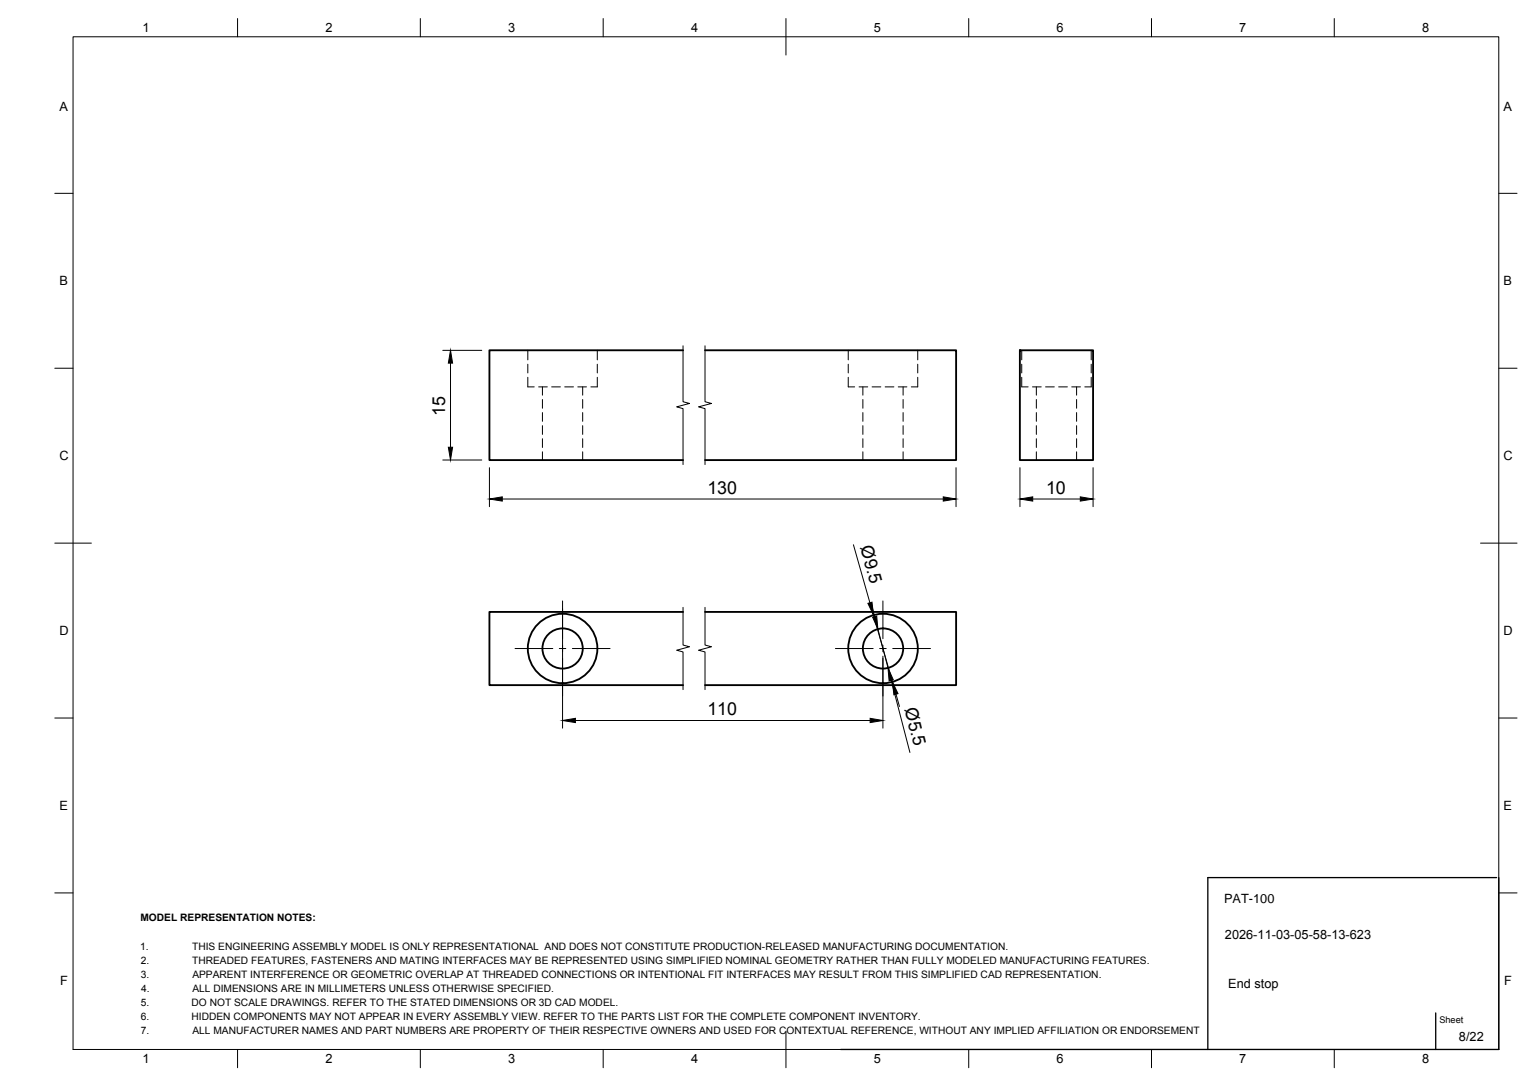
ISO-10303-21;
HEADER;
/* Generated by software containing ST-Developer
 * from STEP Tools, Inc. (www.steptools.com) 
 */

FILE_DESCRIPTION(
/* description */ (''),
/* implementation_level */ '2;1');

FILE_NAME(
/* name */ 'End stop.step',
/* time_stamp */ '2026-10-29T16:43:51-07:00',
/* author */ (''),
/* organization */ (''),
/* preprocessor_version */ 'ST-DEVELOPER v20.2',
/* originating_system */ 'Autodesk Translation Framework v15.17.0.0',
/* authorisation */ '');

FILE_SCHEMA (('AUTOMOTIVE_DESIGN { 1 0 10303 214 3 1 1 }'));
ENDSEC;

DATA;
#10=MECHANICAL_DESIGN_GEOMETRIC_PRESENTATION_REPRESENTATION('',(#369),#10292);
#323=SHAPE_REPRESENTATION_RELATIONSHIP('SRR','None',#10419,#346);
#346=ADVANCED_BREP_SHAPE_REPRESENTATION('',(#391),#10271);
#369=STYLED_ITEM('',(#10621),#391);
#391=MANIFOLD_SOLID_BREP('Body1',#5012);
#449=FACE_BOUND('',#1109,.T.);
#450=FACE_BOUND('',#1112,.T.);
#451=FACE_BOUND('',#1120,.T.);
#452=FACE_BOUND('',#1121,.T.);
#453=FACE_BOUND('',#1123,.T.);
#454=FACE_BOUND('',#1124,.T.);
#566=PLANE('',#5422);
#567=PLANE('',#5427);
#568=PLANE('',#5433);
#569=PLANE('',#5434);
#570=PLANE('',#5435);
#571=PLANE('',#5436);
#572=PLANE('',#5437);
#573=PLANE('',#5438);
#776=FACE_OUTER_BOUND('',#1107,.T.);
#777=FACE_OUTER_BOUND('',#1108,.T.);
#778=FACE_OUTER_BOUND('',#1110,.T.);
#779=FACE_OUTER_BOUND('',#1111,.T.);
#780=FACE_OUTER_BOUND('',#1113,.T.);
#781=FACE_OUTER_BOUND('',#1114,.T.);
#782=FACE_OUTER_BOUND('',#1115,.T.);
#783=FACE_OUTER_BOUND('',#1116,.T.);
#784=FACE_OUTER_BOUND('',#1117,.T.);
#785=FACE_OUTER_BOUND('',#1118,.T.);
#786=FACE_OUTER_BOUND('',#1119,.T.);
#787=FACE_OUTER_BOUND('',#1122,.T.);
#1107=EDGE_LOOP('',(#3729,#3730,#3731,#3732));
#1108=EDGE_LOOP('',(#3733));
#1109=EDGE_LOOP('',(#3734));
#1110=EDGE_LOOP('',(#3735,#3736,#3737,#3738));
#1111=EDGE_LOOP('',(#3739));
#1112=EDGE_LOOP('',(#3740));
#1113=EDGE_LOOP('',(#3741,#3742,#3743,#3744));
#1114=EDGE_LOOP('',(#3745,#3746,#3747,#3748));
#1115=EDGE_LOOP('',(#3749,#3750,#3751,#3752));
#1116=EDGE_LOOP('',(#3753,#3754,#3755,#3756));
#1117=EDGE_LOOP('',(#3757,#3758,#3759,#3760));
#1118=EDGE_LOOP('',(#3761,#3762,#3763,#3764));
#1119=EDGE_LOOP('',(#3765,#3766,#3767,#3768));
#1120=EDGE_LOOP('',(#3769));
#1121=EDGE_LOOP('',(#3770));
#1122=EDGE_LOOP('',(#3771,#3772,#3773,#3774));
#1123=EDGE_LOOP('',(#3775));
#1124=EDGE_LOOP('',(#3776));
#1514=LINE('',#7748,#1906);
#1515=LINE('',#7757,#1907);
#1516=LINE('',#7765,#1908);
#1517=LINE('',#7769,#1909);
#1518=LINE('',#7773,#1910);
#1519=LINE('',#7775,#1911);
#1520=LINE('',#7777,#1912);
#1521=LINE('',#7778,#1913);
#1522=LINE('',#7781,#1914);
#1523=LINE('',#7783,#1915);
#1524=LINE('',#7784,#1916);
#1525=LINE('',#7787,#1917);
#1526=LINE('',#7789,#1918);
#1527=LINE('',#7790,#1919);
#1528=LINE('',#7792,#1920);
#1529=LINE('',#7793,#1921);
#1906=VECTOR('',#6231,0.475);
#1907=VECTOR('',#6242,0.475);
#1908=VECTOR('',#6253,0.275);
#1909=VECTOR('',#6258,0.275);
#1910=VECTOR('',#6261,1.);
#1911=VECTOR('',#6262,1.);
#1912=VECTOR('',#6263,1.);
#1913=VECTOR('',#6264,1.);
#1914=VECTOR('',#6267,1.);
#1915=VECTOR('',#6268,1.);
#1916=VECTOR('',#6269,1.);
#1917=VECTOR('',#6272,1.);
#1918=VECTOR('',#6273,1.);
#1919=VECTOR('',#6274,1.);
#1920=VECTOR('',#6277,1.);
#1921=VECTOR('',#6278,1.);
#2252=CIRCLE('',#5420,0.475);
#2253=CIRCLE('',#5421,0.475);
#2254=CIRCLE('',#5423,0.275);
#2255=CIRCLE('',#5425,0.475);
#2256=CIRCLE('',#5426,0.475);
#2257=CIRCLE('',#5428,0.275);
#2258=CIRCLE('',#5430,0.275);
#2259=CIRCLE('',#5432,0.275);
#2499=VERTEX_POINT('',#7745);
#2500=VERTEX_POINT('',#7747);
#2501=VERTEX_POINT('',#7751);
#2502=VERTEX_POINT('',#7754);
#2503=VERTEX_POINT('',#7756);
#2504=VERTEX_POINT('',#7760);
#2505=VERTEX_POINT('',#7763);
#2506=VERTEX_POINT('',#7767);
#2507=VERTEX_POINT('',#7771);
#2508=VERTEX_POINT('',#7772);
#2509=VERTEX_POINT('',#7774);
#2510=VERTEX_POINT('',#7776);
#2511=VERTEX_POINT('',#7780);
#2512=VERTEX_POINT('',#7782);
#2513=VERTEX_POINT('',#7786);
#2514=VERTEX_POINT('',#7788);
#2955=EDGE_CURVE('',#2499,#2499,#2252,.T.);
#2956=EDGE_CURVE('',#2499,#2500,#1514,.T.);
#2957=EDGE_CURVE('',#2500,#2500,#2253,.T.);
#2958=EDGE_CURVE('',#2501,#2501,#2254,.T.);
#2959=EDGE_CURVE('',#2502,#2502,#2255,.T.);
#2960=EDGE_CURVE('',#2502,#2503,#1515,.T.);
#2961=EDGE_CURVE('',#2503,#2503,#2256,.T.);
#2962=EDGE_CURVE('',#2504,#2504,#2257,.T.);
#2963=EDGE_CURVE('',#2505,#2505,#2258,.T.);
#2964=EDGE_CURVE('',#2505,#2501,#1516,.T.);
#2965=EDGE_CURVE('',#2506,#2506,#2259,.T.);
#2966=EDGE_CURVE('',#2506,#2504,#1517,.T.);
#2967=EDGE_CURVE('',#2507,#2508,#1518,.T.);
#2968=EDGE_CURVE('',#2508,#2509,#1519,.T.);
#2969=EDGE_CURVE('',#2510,#2509,#1520,.T.);
#2970=EDGE_CURVE('',#2507,#2510,#1521,.T.);
#2971=EDGE_CURVE('',#2511,#2507,#1522,.T.);
#2972=EDGE_CURVE('',#2512,#2510,#1523,.T.);
#2973=EDGE_CURVE('',#2511,#2512,#1524,.T.);
#2974=EDGE_CURVE('',#2513,#2511,#1525,.T.);
#2975=EDGE_CURVE('',#2514,#2512,#1526,.T.);
#2976=EDGE_CURVE('',#2513,#2514,#1527,.T.);
#2977=EDGE_CURVE('',#2508,#2513,#1528,.T.);
#2978=EDGE_CURVE('',#2509,#2514,#1529,.T.);
#3729=ORIENTED_EDGE('',*,*,#2955,.F.);
#3730=ORIENTED_EDGE('',*,*,#2956,.T.);
#3731=ORIENTED_EDGE('',*,*,#2957,.F.);
#3732=ORIENTED_EDGE('',*,*,#2956,.F.);
#3733=ORIENTED_EDGE('',*,*,#2955,.T.);
#3734=ORIENTED_EDGE('',*,*,#2958,.F.);
#3735=ORIENTED_EDGE('',*,*,#2959,.F.);
#3736=ORIENTED_EDGE('',*,*,#2960,.T.);
#3737=ORIENTED_EDGE('',*,*,#2961,.F.);
#3738=ORIENTED_EDGE('',*,*,#2960,.F.);
#3739=ORIENTED_EDGE('',*,*,#2959,.T.);
#3740=ORIENTED_EDGE('',*,*,#2962,.F.);
#3741=ORIENTED_EDGE('',*,*,#2963,.F.);
#3742=ORIENTED_EDGE('',*,*,#2964,.T.);
#3743=ORIENTED_EDGE('',*,*,#2958,.T.);
#3744=ORIENTED_EDGE('',*,*,#2964,.F.);
#3745=ORIENTED_EDGE('',*,*,#2965,.F.);
#3746=ORIENTED_EDGE('',*,*,#2966,.T.);
#3747=ORIENTED_EDGE('',*,*,#2962,.T.);
#3748=ORIENTED_EDGE('',*,*,#2966,.F.);
#3749=ORIENTED_EDGE('',*,*,#2967,.T.);
#3750=ORIENTED_EDGE('',*,*,#2968,.T.);
#3751=ORIENTED_EDGE('',*,*,#2969,.F.);
#3752=ORIENTED_EDGE('',*,*,#2970,.F.);
#3753=ORIENTED_EDGE('',*,*,#2971,.T.);
#3754=ORIENTED_EDGE('',*,*,#2970,.T.);
#3755=ORIENTED_EDGE('',*,*,#2972,.F.);
#3756=ORIENTED_EDGE('',*,*,#2973,.F.);
#3757=ORIENTED_EDGE('',*,*,#2974,.T.);
#3758=ORIENTED_EDGE('',*,*,#2973,.T.);
#3759=ORIENTED_EDGE('',*,*,#2975,.F.);
#3760=ORIENTED_EDGE('',*,*,#2976,.F.);
#3761=ORIENTED_EDGE('',*,*,#2977,.T.);
#3762=ORIENTED_EDGE('',*,*,#2976,.T.);
#3763=ORIENTED_EDGE('',*,*,#2978,.F.);
#3764=ORIENTED_EDGE('',*,*,#2968,.F.);
#3765=ORIENTED_EDGE('',*,*,#2978,.T.);
#3766=ORIENTED_EDGE('',*,*,#2975,.T.);
#3767=ORIENTED_EDGE('',*,*,#2972,.T.);
#3768=ORIENTED_EDGE('',*,*,#2969,.T.);
#3769=ORIENTED_EDGE('',*,*,#2957,.T.);
#3770=ORIENTED_EDGE('',*,*,#2961,.T.);
#3771=ORIENTED_EDGE('',*,*,#2977,.F.);
#3772=ORIENTED_EDGE('',*,*,#2967,.F.);
#3773=ORIENTED_EDGE('',*,*,#2971,.F.);
#3774=ORIENTED_EDGE('',*,*,#2974,.F.);
#3775=ORIENTED_EDGE('',*,*,#2963,.T.);
#3776=ORIENTED_EDGE('',*,*,#2965,.T.);
#4663=CYLINDRICAL_SURFACE('',#5419,0.475);
#4664=CYLINDRICAL_SURFACE('',#5424,0.475);
#4665=CYLINDRICAL_SURFACE('',#5429,0.275);
#4666=CYLINDRICAL_SURFACE('',#5431,0.275);
#4785=ADVANCED_FACE('',(#776),#4663,.F.);
#4786=ADVANCED_FACE('',(#777,#449),#566,.T.);
#4787=ADVANCED_FACE('',(#778),#4664,.F.);
#4788=ADVANCED_FACE('',(#779,#450),#567,.T.);
#4789=ADVANCED_FACE('',(#780),#4665,.F.);
#4790=ADVANCED_FACE('',(#781),#4666,.F.);
#4791=ADVANCED_FACE('',(#782),#568,.T.);
#4792=ADVANCED_FACE('',(#783),#569,.T.);
#4793=ADVANCED_FACE('',(#784),#570,.T.);
#4794=ADVANCED_FACE('',(#785),#571,.T.);
#4795=ADVANCED_FACE('',(#786,#451,#452),#572,.T.);
#4796=ADVANCED_FACE('',(#787,#453,#454),#573,.F.);
#5012=CLOSED_SHELL('',(#4785,#4786,#4787,#4788,#4789,#4790,#4791,#4792,
#4793,#4794,#4795,#4796));
#5418=AXIS2_PLACEMENT_3D('',#7743,#6225,#6226);
#5419=AXIS2_PLACEMENT_3D('',#7744,#6227,#6228);
#5420=AXIS2_PLACEMENT_3D('',#7746,#6229,#6230);
#5421=AXIS2_PLACEMENT_3D('',#7749,#6232,#6233);
#5422=AXIS2_PLACEMENT_3D('',#7750,#6234,#6235);
#5423=AXIS2_PLACEMENT_3D('',#7752,#6236,#6237);
#5424=AXIS2_PLACEMENT_3D('',#7753,#6238,#6239);
#5425=AXIS2_PLACEMENT_3D('',#7755,#6240,#6241);
#5426=AXIS2_PLACEMENT_3D('',#7758,#6243,#6244);
#5427=AXIS2_PLACEMENT_3D('',#7759,#6245,#6246);
#5428=AXIS2_PLACEMENT_3D('',#7761,#6247,#6248);
#5429=AXIS2_PLACEMENT_3D('',#7762,#6249,#6250);
#5430=AXIS2_PLACEMENT_3D('',#7764,#6251,#6252);
#5431=AXIS2_PLACEMENT_3D('',#7766,#6254,#6255);
#5432=AXIS2_PLACEMENT_3D('',#7768,#6256,#6257);
#5433=AXIS2_PLACEMENT_3D('',#7770,#6259,#6260);
#5434=AXIS2_PLACEMENT_3D('',#7779,#6265,#6266);
#5435=AXIS2_PLACEMENT_3D('',#7785,#6270,#6271);
#5436=AXIS2_PLACEMENT_3D('',#7791,#6275,#6276);
#5437=AXIS2_PLACEMENT_3D('',#7794,#6279,#6280);
#5438=AXIS2_PLACEMENT_3D('',#7795,#6281,#6282);
#6225=DIRECTION('axis',(0.,0.,1.));
#6226=DIRECTION('refdir',(1.,0.,0.));
#6227=DIRECTION('center_axis',(0.,0.,1.));
#6228=DIRECTION('ref_axis',(1.,0.,0.));
#6229=DIRECTION('center_axis',(0.,0.,1.));
#6230=DIRECTION('ref_axis',(1.,0.,0.));
#6231=DIRECTION('',(0.,0.,1.));
#6232=DIRECTION('center_axis',(0.,0.,-1.));
#6233=DIRECTION('ref_axis',(1.,0.,0.));
#6234=DIRECTION('center_axis',(0.,0.,1.));
#6235=DIRECTION('ref_axis',(1.,0.,0.));
#6236=DIRECTION('center_axis',(0.,0.,1.));
#6237=DIRECTION('ref_axis',(1.,0.,0.));
#6238=DIRECTION('center_axis',(0.,0.,1.));
#6239=DIRECTION('ref_axis',(1.,0.,0.));
#6240=DIRECTION('center_axis',(0.,0.,1.));
#6241=DIRECTION('ref_axis',(1.,0.,0.));
#6242=DIRECTION('',(0.,0.,1.));
#6243=DIRECTION('center_axis',(0.,0.,-1.));
#6244=DIRECTION('ref_axis',(1.,0.,0.));
#6245=DIRECTION('center_axis',(0.,0.,1.));
#6246=DIRECTION('ref_axis',(1.,0.,0.));
#6247=DIRECTION('center_axis',(0.,0.,1.));
#6248=DIRECTION('ref_axis',(1.,0.,0.));
#6249=DIRECTION('center_axis',(0.,0.,1.));
#6250=DIRECTION('ref_axis',(1.,0.,0.));
#6251=DIRECTION('center_axis',(0.,0.,1.));
#6252=DIRECTION('ref_axis',(1.,0.,0.));
#6253=DIRECTION('',(0.,0.,1.));
#6254=DIRECTION('center_axis',(0.,0.,1.));
#6255=DIRECTION('ref_axis',(1.,0.,0.));
#6256=DIRECTION('center_axis',(0.,0.,1.));
#6257=DIRECTION('ref_axis',(1.,0.,0.));
#6258=DIRECTION('',(0.,0.,1.));
#6259=DIRECTION('center_axis',(0.,1.,0.));
#6260=DIRECTION('ref_axis',(-1.,0.,0.));
#6261=DIRECTION('',(-1.,0.,0.));
#6262=DIRECTION('',(0.,0.,1.));
#6263=DIRECTION('',(-1.,0.,0.));
#6264=DIRECTION('',(0.,0.,1.));
#6265=DIRECTION('center_axis',(1.,0.,0.));
#6266=DIRECTION('ref_axis',(0.,1.,0.));
#6267=DIRECTION('',(0.,1.,0.));
#6268=DIRECTION('',(0.,1.,0.));
#6269=DIRECTION('',(0.,0.,1.));
#6270=DIRECTION('center_axis',(0.,-1.,0.));
#6271=DIRECTION('ref_axis',(1.,0.,0.));
#6272=DIRECTION('',(1.,0.,0.));
#6273=DIRECTION('',(1.,0.,0.));
#6274=DIRECTION('',(0.,0.,1.));
#6275=DIRECTION('center_axis',(-1.,0.,0.));
#6276=DIRECTION('ref_axis',(0.,-1.,0.));
#6277=DIRECTION('',(0.,-1.,0.));
#6278=DIRECTION('',(0.,-1.,0.));
#6279=DIRECTION('center_axis',(0.,0.,1.));
#6280=DIRECTION('ref_axis',(1.,0.,0.));
#6281=DIRECTION('center_axis',(0.,0.,1.));
#6282=DIRECTION('ref_axis',(1.,0.,0.));
#7743=CARTESIAN_POINT('',(0.,0.,0.));
#7744=CARTESIAN_POINT('Origin',(3.5,-5.5,2.));
#7745=CARTESIAN_POINT('',(3.025,-5.5,2.));
#7746=CARTESIAN_POINT('Origin',(3.5,-5.5,2.));
#7747=CARTESIAN_POINT('',(3.025,-5.5,2.5));
#7748=CARTESIAN_POINT('',(3.025,-5.5,2.));
#7749=CARTESIAN_POINT('Origin',(3.5,-5.5,2.5));
#7750=CARTESIAN_POINT('Origin',(3.5,-5.5,2.));
#7751=CARTESIAN_POINT('',(3.225,-5.5,2.));
#7752=CARTESIAN_POINT('Origin',(3.5,-5.5,2.));
#7753=CARTESIAN_POINT('Origin',(3.5,5.5,2.));
#7754=CARTESIAN_POINT('',(3.025,5.5,2.));
#7755=CARTESIAN_POINT('Origin',(3.5,5.5,2.));
#7756=CARTESIAN_POINT('',(3.025,5.5,2.5));
#7757=CARTESIAN_POINT('',(3.025,5.5,2.));
#7758=CARTESIAN_POINT('Origin',(3.5,5.5,2.5));
#7759=CARTESIAN_POINT('Origin',(3.5,5.5,2.));
#7760=CARTESIAN_POINT('',(3.225,5.5,2.));
#7761=CARTESIAN_POINT('Origin',(3.5,5.5,2.));
#7762=CARTESIAN_POINT('Origin',(3.5,-5.5,0.9));
#7763=CARTESIAN_POINT('',(3.225,-5.5,1.));
#7764=CARTESIAN_POINT('Origin',(3.5,-5.5,1.));
#7765=CARTESIAN_POINT('',(3.225,-5.5,0.9));
#7766=CARTESIAN_POINT('Origin',(3.5,5.5,0.9));
#7767=CARTESIAN_POINT('',(3.225,5.5,1.));
#7768=CARTESIAN_POINT('Origin',(3.5,5.5,1.));
#7769=CARTESIAN_POINT('',(3.225,5.5,0.9));
#7770=CARTESIAN_POINT('Origin',(4.,6.5,1.));
#7771=CARTESIAN_POINT('',(4.,6.5,1.));
#7772=CARTESIAN_POINT('',(3.,6.5,1.));
#7773=CARTESIAN_POINT('',(4.,6.5,1.));
#7774=CARTESIAN_POINT('',(3.,6.5,2.5));
#7775=CARTESIAN_POINT('',(3.,6.5,1.));
#7776=CARTESIAN_POINT('',(4.,6.5,2.5));
#7777=CARTESIAN_POINT('',(4.,6.5,2.5));
#7778=CARTESIAN_POINT('',(4.,6.5,1.));
#7779=CARTESIAN_POINT('Origin',(4.,-6.5,1.));
#7780=CARTESIAN_POINT('',(4.,-6.5,1.));
#7781=CARTESIAN_POINT('',(4.,-6.5,1.));
#7782=CARTESIAN_POINT('',(4.,-6.5,2.5));
#7783=CARTESIAN_POINT('',(4.,-6.5,2.5));
#7784=CARTESIAN_POINT('',(4.,-6.5,1.));
#7785=CARTESIAN_POINT('Origin',(3.,-6.5,1.));
#7786=CARTESIAN_POINT('',(3.,-6.5,1.));
#7787=CARTESIAN_POINT('',(3.,-6.5,1.));
#7788=CARTESIAN_POINT('',(3.,-6.5,2.5));
#7789=CARTESIAN_POINT('',(3.,-6.5,2.5));
#7790=CARTESIAN_POINT('',(3.,-6.5,1.));
#7791=CARTESIAN_POINT('Origin',(3.,6.5,1.));
#7792=CARTESIAN_POINT('',(3.,6.5,1.));
#7793=CARTESIAN_POINT('',(3.,6.5,2.5));
#7794=CARTESIAN_POINT('Origin',(3.5,0.,2.5));
#7795=CARTESIAN_POINT('Origin',(3.5,0.,1.));
#10243=UNCERTAINTY_MEASURE_WITH_UNIT(LENGTH_MEASURE(0.001),#10293,
'DISTANCE_ACCURACY_VALUE',
'Maximum model space distance between geometric entities at asserted c
onnectivities');
#10264=UNCERTAINTY_MEASURE_WITH_UNIT(LENGTH_MEASURE(0.001),#10293,
'DISTANCE_ACCURACY_VALUE',
'Maximum model space distance between geometric entities at asserted c
onnectivities');
#10271=(
GEOMETRIC_REPRESENTATION_CONTEXT(3)
GLOBAL_UNCERTAINTY_ASSIGNED_CONTEXT((#10243))
GLOBAL_UNIT_ASSIGNED_CONTEXT((#10293,#10295,#10296))
REPRESENTATION_CONTEXT('','3D')
);
#10292=(
GEOMETRIC_REPRESENTATION_CONTEXT(3)
GLOBAL_UNCERTAINTY_ASSIGNED_CONTEXT((#10264))
GLOBAL_UNIT_ASSIGNED_CONTEXT((#10293,#10295,#10296))
REPRESENTATION_CONTEXT('','3D')
);
#10293=(
LENGTH_UNIT()
NAMED_UNIT(*)
SI_UNIT(.CENTI.,.METRE.)
);
#10295=(
NAMED_UNIT(*)
PLANE_ANGLE_UNIT()
SI_UNIT($,.RADIAN.)
);
#10296=(
NAMED_UNIT(*)
SI_UNIT($,.STERADIAN.)
SOLID_ANGLE_UNIT()
);
#10303=SHAPE_DEFINITION_REPRESENTATION(#10330,#10419);
#10330=PRODUCT_DEFINITION_SHAPE('',$,#10447);
#10419=SHAPE_REPRESENTATION('',(#5418),#10271);
#10440=PRODUCT_DEFINITION_CONTEXT('part definition',#10523,'design');
#10447=PRODUCT_DEFINITION('End stop','End stop',#10474,#10440);
#10474=PRODUCT_DEFINITION_FORMATION('',$,#10531);
#10523=APPLICATION_CONTEXT(
'Core Data for Automotive Mechanical Design Process');
#10524=PRODUCT_CONTEXT('part definition',#10523,'mechanical');
#10531=PRODUCT('End stop','End stop','End stop',(#10524));
#10615=COLOUR_RGB('Sky Blue',0.24,0.69,0.87);
#10616=FILL_AREA_STYLE_COLOUR('',#10615);
#10617=FILL_AREA_STYLE('',(#10616));
#10618=SURFACE_STYLE_FILL_AREA(#10617);
#10619=SURFACE_SIDE_STYLE('',(#10618));
#10620=SURFACE_STYLE_USAGE(.BOTH.,#10619);
#10621=PRESENTATION_STYLE_ASSIGNMENT((#10620));
ENDSEC;
END-ISO-10303-21;
